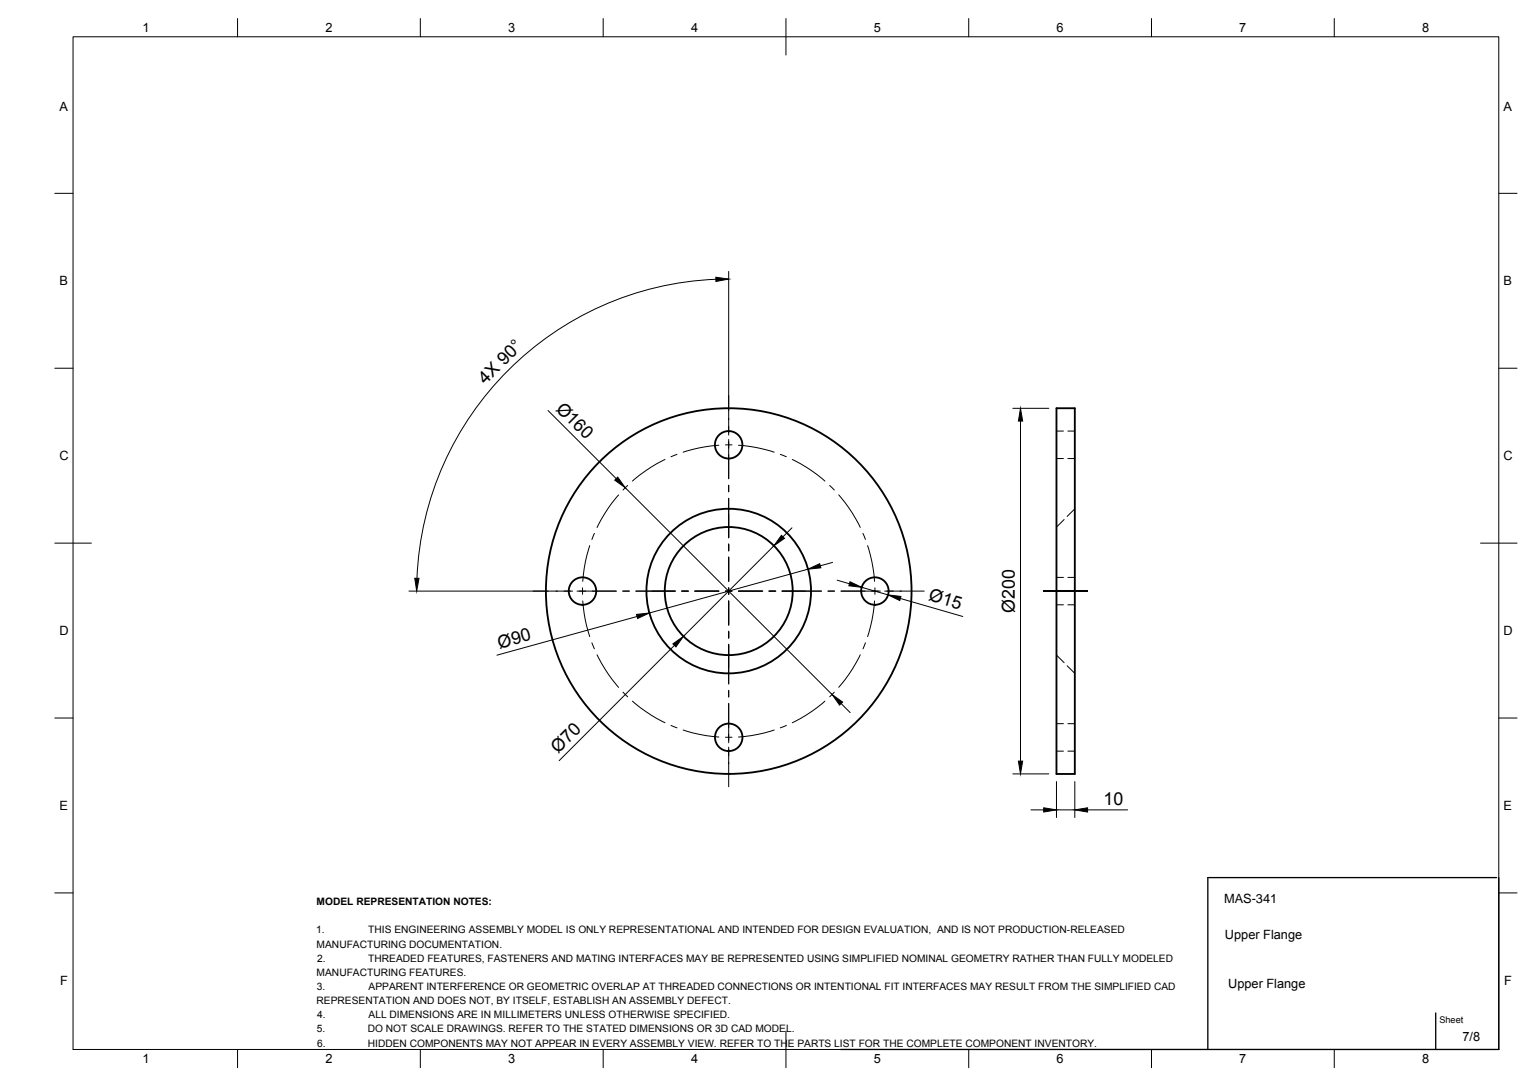
ISO-10303-21;
HEADER;
FILE_DESCRIPTION (('STEP AP214'),
    '1' );
FILE_NAME ('Upper Flange.step',
    '2026-10-08T00:39:10',
    ( '' ),
    ( '' ),
    'SwSTEP 2.0',
    'SolidWorks 2025',
    '' );
FILE_SCHEMA (( 'AUTOMOTIVE_DESIGN' ));
ENDSEC;

DATA;
#46=DIRECTION ( 'NONE',  ( 0.000000000000000000, 1.000000000000000000, 0.000000000000000000 ) ) ;
#104=VECTOR ( 'NONE', #2637, 1000.000000000000000 ) ;
#106=FACE_OUTER_BOUND ( 'NONE', #19908, .T. ) ;
#339=FACE_OUTER_BOUND ( 'NONE', #16289, .T. ) ;
#345=VERTEX_POINT ( 'NONE', #11779 ) ;
#367=EDGE_LOOP ( 'NONE', ( #4657, #4676 ) ) ;
#371=VERTEX_POINT ( 'NONE', #9014 ) ;
#373=ADVANCED_FACE ( 'NONE', ( #2893 ), #13929, .F. ) ;
#378=DIRECTION ( 'NONE',  ( -0.000000000000000000, -1.000000000000000000, -0.000000000000000000 ) ) ;
#387=CARTESIAN_POINT ( 'NONE',  ( -109.9999999999983515, 285.0000000000000568, 92.50000000000004263 ) ) ;
#392=ORIENTED_EDGE ( 'NONE', *, *, #15866, .T. ) ;
#411=DIRECTION ( 'NONE',  ( 0.000000000000000000, 0.000000000000000000, -1.000000000000000000 ) ) ;
#419=PLANE ( 'NONE',  #4671 ) ;
#422=CARTESIAN_POINT ( 'NONE',  ( -110.0000000000000142, 285.0000000000000568, -82.50000000000001421 ) ) ;
#511=DIRECTION ( 'NONE',  ( 0.000000000000000000, 1.000000000000000000, 0.000000000000000000 ) ) ;
#541=VERTEX_POINT ( 'NONE', #10137 ) ;
#552=EDGE_LOOP ( 'NONE', ( #7577, #5145, #8695, #8498 ) ) ;
#564=DIRECTION ( 'NONE',  ( -0.000000000000000000, -1.000000000000000000, -0.000000000000000000 ) ) ;
#565=DIRECTION ( 'NONE',  ( -0.000000000000000000, -1.000000000000000000, -0.000000000000000000 ) ) ;
#609=CIRCLE ( 'NONE', #7461, 34.99999999999997868 ) ;
#638=ORIENTED_EDGE ( 'NONE', *, *, #4760, .F. ) ;
#642=CARTESIAN_POINT ( 'NONE',  ( -110.0000000000000142, 275.0000000000000000, 5.000000000000000888 ) ) ;
#648=VERTEX_POINT ( 'NONE', #17925 ) ;
#660=EDGE_CURVE ( 'NONE', #17410, #15549, #8916, .T. ) ;
#668=PRODUCT_DEFINITION_CONTEXT ( 'detailed design', #4634, 'design' ) ;
#671=PRODUCT_DEFINITION_FORMATION_WITH_SPECIFIED_SOURCE ( 'ANY', '', #15700, .NOT_KNOWN. ) ;
#676=ORIENTED_EDGE ( 'NONE', *, *, #9749, .T. ) ;
#775=AXIS2_PLACEMENT_3D ( 'NONE', #10807, #9387, #14194 ) ;
#811=CIRCLE ( 'NONE', #18457, 99.99999999999997158 ) ;
#815=CARTESIAN_POINT ( 'NONE',  ( -29.99999999999887379, 275.0000000000000000, 4.999999999999158007 ) ) ;
#883=ORIENTED_EDGE ( 'NONE', *, *, #14292, .T. ) ;
#1036=AXIS2_PLACEMENT_3D ( 'NONE', #12711, #18869, #17440 ) ;
#1094=EDGE_CURVE ( 'NONE', #541, #1941, #19405, .T. ) ;
#1096=DIRECTION ( 'NONE',  ( -0.000000000000000000, -1.000000000000000000, -0.000000000000000000 ) ) ;
#1099=EDGE_CURVE ( 'NONE', #16204, #18358, #3152, .T. ) ;
#1141=EDGE_LOOP ( 'NONE', ( #1644, #11755 ) ) ;
#1161=ORIENTED_EDGE ( 'NONE', *, *, #1765, .F. ) ;
#1186=MANIFOLD_SOLID_BREP ( 'Chamfer1', #7388 ) ;
#1187=VERTEX_POINT ( 'NONE', #19014 ) ;
#1382=VECTOR ( 'NONE', #13012, 1000.000000000000000 ) ;
#1402=EDGE_LOOP ( 'NONE', ( #11155, #2446, #12157, #14344 ) ) ;
#1517=AXIS2_PLACEMENT_3D ( 'NONE', #15686, #15576, #15255 ) ;
#1539=ORIENTED_EDGE ( 'NONE', *, *, #14292, .F. ) ;
#1564=CARTESIAN_POINT ( 'NONE',  ( -29.99999999999887379, 285.0000000000000568, 4.999999999999158007 ) ) ;
#1644=ORIENTED_EDGE ( 'NONE', *, *, #9146, .T. ) ;
#1750=CARTESIAN_POINT ( 'NONE',  ( -110.0000000000000142, 285.0000000000000568, 5.000000000000000888 ) ) ;
#1765=EDGE_CURVE ( 'NONE', #16453, #5784, #19740, .T. ) ;
#1868=FACE_BOUND ( 'NONE', #4582, .T. ) ;
#1922=FILL_AREA_STYLE ('',( #15934 ) ) ;
#1941=VERTEX_POINT ( 'NONE', #1953 ) ;
#1953=CARTESIAN_POINT ( 'NONE',  ( -110.0000000000000142, 285.0000000000000568, 50.00000000000000000 ) ) ;
#1971=PRODUCT_CONTEXT ( 'NONE', #13758, 'mechanical' ) ;
#1976=FACE_OUTER_BOUND ( 'NONE', #19531, .T. ) ;
#2046=DIRECTION ( 'NONE',  ( 0.000000000000000000, 0.000000000000000000, 1.000000000000000000 ) ) ;
#2093=COLOUR_RGB ( '', 0.40784314, 0.44705882, 0.49803922) ;
#2165=FACE_BOUND ( 'NONE', #2281, .T. ) ;
#2279=FACE_BOUND ( 'NONE', #10646, .T. ) ;
#2281=EDGE_LOOP ( 'NONE', ( #15820, #17001 ) ) ;
#2293=CYLINDRICAL_SURFACE ( 'NONE', #10703, 99.99999999999997158 ) ;
#2388=EDGE_CURVE ( 'NONE', #13281, #345, #2976, .T. ) ;
#2425=LINE ( 'NONE', #2517, #20217 ) ;
#2437=ORIENTED_EDGE ( 'NONE', *, *, #13531, .F. ) ;
#2446=ORIENTED_EDGE ( 'NONE', *, *, #11970, .F. ) ;
#2479=EDGE_LOOP ( 'NONE', ( #13804, #13370 ) ) ;
#2509=CONICAL_SURFACE ( 'NONE', #10337, 34.99999999999997868, 0.7853981633974521648 ) ;
#2517=CARTESIAN_POINT ( 'NONE',  ( -109.9999999999983515, 285.0000000000000568, 92.50000000000004263 ) ) ;
#2529=CARTESIAN_POINT ( 'NONE',  ( -29.99999999999887379, 285.0000000000000568, -2.500000000000847766 ) ) ;
#2548=CARTESIAN_POINT ( 'NONE',  ( -29.99999999999887379, 275.0000000000000000, 12.49999999999916511 ) ) ;
#2559=ORIENTED_EDGE ( 'NONE', *, *, #8365, .F. ) ;
#2600=ORIENTED_EDGE ( 'NONE', *, *, #11970, .T. ) ;
#2618=DIRECTION ( 'NONE',  ( 0.000000000000000000, 1.000000000000000000, 0.000000000000000000 ) ) ;
#2624=CIRCLE ( 'NONE', #17073, 7.500000000000020428 ) ;
#2637=DIRECTION ( 'NONE',  ( 0.000000000000000000, 0.7071067811865447972, 0.7071067811865502373 ) ) ;
#2651=CARTESIAN_POINT ( 'NONE',  ( -109.9999999999983515, 285.0000000000000568, 85.00000000000001421 ) ) ;
#2681=LINE ( 'NONE', #13204, #19215 ) ;
#2712=ORIENTED_EDGE ( 'NONE', *, *, #660, .F. ) ;
#2730=DIRECTION ( 'NONE',  ( 0.000000000000000000, 1.000000000000000000, 0.000000000000000000 ) ) ;
#2793=VERTEX_POINT ( 'NONE', #13529 ) ;
#2814=ORIENTED_EDGE ( 'NONE', *, *, #15802, .T. ) ;
#2893=FACE_OUTER_BOUND ( 'NONE', #3242, .T. ) ;
#2937=AXIS2_PLACEMENT_3D ( 'NONE', #11804, #7124, #5792 ) ;
#2976=CIRCLE ( 'NONE', #4279, 7.500000000000020428 ) ;
#2996=EDGE_LOOP ( 'NONE', ( #14290, #392, #6277, #2437 ) ) ;
#3007=DIRECTION ( 'NONE',  ( -0.000000000000000000, -1.000000000000000000, -0.000000000000000000 ) ) ;
#3152=LINE ( 'NONE', #17171, #15816 ) ;
#3169=CARTESIAN_POINT ( 'NONE',  ( -189.9999999999988916, 285.0000000000000568, 5.000000000000268230 ) ) ;
#3228=VECTOR ( 'NONE', #565, 1000.000000000000000 ) ;
#3242=EDGE_LOOP ( 'NONE', ( #10222, #5250, #13945, #15544 ) ) ;
#3422=( GEOMETRIC_REPRESENTATION_CONTEXT ( 3 ) GLOBAL_UNCERTAINTY_ASSIGNED_CONTEXT ( ( #12118 ) ) GLOBAL_UNIT_ASSIGNED_CONTEXT ( ( #18810, #17376, #7944 ) ) REPRESENTATION_CONTEXT ( 'NONE', 'WORKASPACE' ) );
#3444=VERTEX_POINT ( 'NONE', #4937 ) ;
#3478=CARTESIAN_POINT ( 'NONE',  ( -110.0000000000000142, 285.0000000000000568, 5.000000000000000888 ) ) ;
#3524=PRODUCT_DEFINITION ( 'UNKNOWN', '', #671, #668 ) ;
#3532=CARTESIAN_POINT ( 'NONE',  ( -110.0000000000000142, 285.0000000000000568, -67.49999999999997158 ) ) ;
#3541=VECTOR ( 'NONE', #5142, 1000.000000000000000 ) ;
#3710=CIRCLE ( 'NONE', #16124, 7.500000000000007105 ) ;
#3768=CARTESIAN_POINT ( 'NONE',  ( -110.0000000000000142, 275.0000000000000568, 5.000000000000000888 ) ) ;
#3770=LINE ( 'NONE', #5415, #5109 ) ;
#3771=FACE_OUTER_BOUND ( 'NONE', #14291, .T. ) ;
#3784=FACE_BOUND ( 'NONE', #10674, .T. ) ;
#3787=DIRECTION ( 'NONE',  ( 0.000000000000000000, 1.000000000000000000, 0.000000000000000000 ) ) ;
#3799=DIRECTION ( 'NONE',  ( 0.000000000000000000, 1.000000000000000000, 0.000000000000000000 ) ) ;
#3801=EDGE_LOOP ( 'NONE', ( #2712, #9678, #676, #12389 ) ) ;
#3870=EDGE_CURVE ( 'NONE', #7406, #3444, #2624, .T. ) ;
#3909=DIRECTION ( 'NONE',  ( 0.000000000000000000, 0.000000000000000000, 1.000000000000000000 ) ) ;
#4075=CARTESIAN_POINT ( 'NONE',  ( -110.0000000000000142, 275.0000000000000568, 5.000000000000000888 ) ) ;
#4084=AXIS2_PLACEMENT_3D ( 'NONE', #19276, #11584, #14458 ) ;
#4118=EDGE_CURVE ( 'NONE', #16923, #16598, #15430, .T. ) ;
#4156=DIRECTION ( 'NONE',  ( 0.000000000000000000, 0.000000000000000000, 1.000000000000000000 ) ) ;
#4173=ORIENTED_EDGE ( 'NONE', *, *, #4760, .T. ) ;
#4279=AXIS2_PLACEMENT_3D ( 'NONE', #10191, #13349, #11809 ) ;
#4294=CARTESIAN_POINT ( 'NONE',  ( -110.0000000000000142, 285.0000000000000568, 5.000000000000000888 ) ) ;
#4344=CIRCLE ( 'NONE', #13475, 45.00000000000001421 ) ;
#4536=CARTESIAN_POINT ( 'NONE',  ( -109.9999999999983515, 285.0000000000000568, 85.00000000000001421 ) ) ;
#4582=EDGE_LOOP ( 'NONE', ( #7260, #4173 ) ) ;
#4624=ORIENTED_EDGE ( 'NONE', *, *, #12645, .F. ) ;
#4634=APPLICATION_CONTEXT ( 'automotive_design' ) ;
#4649=CARTESIAN_POINT ( 'NONE',  ( -189.9999999999988916, 285.0000000000000568, 5.000000000000268230 ) ) ;
#4657=ORIENTED_EDGE ( 'NONE', *, *, #12645, .T. ) ;
#4671=AXIS2_PLACEMENT_3D ( 'NONE', #1750, #7984, #18010 ) ;
#4676=ORIENTED_EDGE ( 'NONE', *, *, #16658, .T. ) ;
#4760=EDGE_CURVE ( 'NONE', #19487, #18358, #3710, .T. ) ;
#4937=CARTESIAN_POINT ( 'NONE',  ( -110.0000000000000142, 275.0000000000000000, -82.50000000000001421 ) ) ;
#4981=ADVANCED_FACE ( 'NONE', ( #17188 ), #5113, .F. ) ;
#4983=CARTESIAN_POINT ( 'NONE',  ( -110.0000000000000142, 275.0000000000000000, -94.99999999999997158 ) ) ;
#5040=LINE ( 'NONE', #422, #3541 ) ;
#5097=SURFACE_STYLE_USAGE ( .BOTH. , #11114 ) ;
#5109=VECTOR ( 'NONE', #20024, 1000.000000000000000 ) ;
#5113=CYLINDRICAL_SURFACE ( 'NONE', #14164, 7.500000000000003553 ) ;
#5142=DIRECTION ( 'NONE',  ( -0.000000000000000000, -1.000000000000000000, -0.000000000000000000 ) ) ;
#5145=ORIENTED_EDGE ( 'NONE', *, *, #4118, .T. ) ;
#5160=CIRCLE ( 'NONE', #19199, 7.500000000000020428 ) ;
#5190=ORIENTED_EDGE ( 'NONE', *, *, #9146, .F. ) ;
#5191=ORIENTED_EDGE ( 'NONE', *, *, #3870, .F. ) ;
#5248=PLANE ( 'NONE',  #16148 ) ;
#5250=ORIENTED_EDGE ( 'NONE', *, *, #7228, .T. ) ;
#5305=DIRECTION ( 'NONE',  ( 0.000000000000000000, 0.000000000000000000, -1.000000000000000000 ) ) ;
#5308=CIRCLE ( 'NONE', #16727, 34.99999999999997868 ) ;
#5326=FACE_OUTER_BOUND ( 'NONE', #1402, .T. ) ;
#5415=CARTESIAN_POINT ( 'NONE',  ( -110.0000000000000000, 285.0000000000000568, 104.9999999999999858 ) ) ;
#5449=DIRECTION ( 'NONE',  ( 0.000000000000000000, 1.000000000000000000, 0.000000000000000000 ) ) ;
#5496=CARTESIAN_POINT ( 'NONE',  ( -110.0000000000000000, 285.0000000000000568, 104.9999999999999858 ) ) ;
#5523=DIRECTION ( 'NONE',  ( 0.000000000000000000, 1.000000000000000000, 0.000000000000000000 ) ) ;
#5549=CIRCLE ( 'NONE', #2937, 99.99999999999997158 ) ;
#5562=DIRECTION ( 'NONE',  ( 0.000000000000000000, 0.000000000000000000, 1.000000000000000000 ) ) ;
#5573=AXIS2_PLACEMENT_3D ( 'NONE', #19141, #7774, #411 ) ;
#5721=DIRECTION ( 'NONE',  ( 0.000000000000000000, 0.000000000000000000, 1.000000000000000000 ) ) ;
#5784=VERTEX_POINT ( 'NONE', #12929 ) ;
#5792=DIRECTION ( 'NONE',  ( 0.000000000000000000, 0.000000000000000000, 1.000000000000000000 ) ) ;
#6058=CARTESIAN_POINT ( 'NONE',  ( -109.9999999999983515, 275.0000000000000000, 85.00000000000001421 ) ) ;
#6078=FACE_OUTER_BOUND ( 'NONE', #14539, .T. ) ;
#6091=ORIENTED_EDGE ( 'NONE', *, *, #11766, .T. ) ;
#6231=AXIS2_PLACEMENT_3D ( 'NONE', #4536, #3007, #7696 ) ;
#6277=ORIENTED_EDGE ( 'NONE', *, *, #13465, .F. ) ;
#6401=ORIENTED_EDGE ( 'NONE', *, *, #12375, .T. ) ;
#6416=CARTESIAN_POINT ( 'NONE',  ( -110.0000000000000142, 275.0000000000000000, -29.99999999999998224 ) ) ;
#6474=ORIENTED_EDGE ( 'NONE', *, *, #11766, .F. ) ;
#6485=VECTOR ( 'NONE', #18378, 1000.000000000000000 ) ;
#6580=ORIENTED_EDGE ( 'NONE', *, *, #4118, .F. ) ;
#6660=CYLINDRICAL_SURFACE ( 'NONE', #17825, 7.500000000000020428 ) ;
#6747=DIRECTION ( 'NONE',  ( -0.000000000000000000, -1.000000000000000000, -0.000000000000000000 ) ) ;
#6754=DIRECTION ( 'NONE',  ( 0.000000000000000000, 0.000000000000000000, 1.000000000000000000 ) ) ;
#6903=CARTESIAN_POINT ( 'NONE',  ( -189.9999999999988916, 275.0000000000000000, 5.000000000000268230 ) ) ;
#7007=EDGE_CURVE ( 'NONE', #16598, #16923, #19661, .T. ) ;
#7072=AXIS2_PLACEMENT_3D ( 'NONE', #7625, #20211, #12433 ) ;
#7093=EDGE_CURVE ( 'NONE', #16460, #371, #5308, .T. ) ;
#7124=DIRECTION ( 'NONE',  ( 0.000000000000000000, 1.000000000000000000, 0.000000000000000000 ) ) ;
#7142=LINE ( 'NONE', #13361, #104 ) ;
#7221=DIRECTION ( 'NONE',  ( -0.000000000000000000, -1.000000000000000000, -0.000000000000000000 ) ) ;
#7228=EDGE_CURVE ( 'NONE', #11511, #19487, #13104, .T. ) ;
#7231=CYLINDRICAL_SURFACE ( 'NONE', #16232, 7.500000000000003553 ) ;
#7260=ORIENTED_EDGE ( 'NONE', *, *, #17492, .T. ) ;
#7303=DIRECTION ( 'NONE',  ( 0.000000000000000000, 1.000000000000000000, 0.000000000000000000 ) ) ;
#7388=CLOSED_SHELL ( 'NONE', ( #11718, #16256, #18901, #373, #9034, #19166, #15927, #14415, #17648, #15605, #19262, #10516, #4981, #16900 ) ) ;
#7406=VERTEX_POINT ( 'NONE', #11049 ) ;
#7461=AXIS2_PLACEMENT_3D ( 'NONE', #15313, #9283, #14193 ) ;
#7525=CARTESIAN_POINT ( 'NONE',  ( -189.9999999999988916, 285.0000000000000568, -2.499999999999734879 ) ) ;
#7577=ORIENTED_EDGE ( 'NONE', *, *, #9978, .F. ) ;
#7617=ORIENTED_EDGE ( 'NONE', *, *, #18627, .T. ) ;
#7625=CARTESIAN_POINT ( 'NONE',  ( -29.99999999999887379, 285.0000000000000568, 4.999999999999158007 ) ) ;
#7672=CYLINDRICAL_SURFACE ( 'NONE', #11118, 99.99999999999997158 ) ;
#7696=DIRECTION ( 'NONE',  ( 0.000000000000000000, 0.000000000000000000, -1.000000000000000000 ) ) ;
#7711=CIRCLE ( 'NONE', #7072, 7.500000000000007105 ) ;
#7774=DIRECTION ( 'NONE',  ( -0.000000000000000000, -1.000000000000000000, -0.000000000000000000 ) ) ;
#7779=DIRECTION ( 'NONE',  ( 0.000000000000000000, 1.000000000000000000, 0.000000000000000000 ) ) ;
#7812=CIRCLE ( 'NONE', #9765, 7.500000000000020428 ) ;
#7823=ORIENTED_EDGE ( 'NONE', *, *, #9670, .T. ) ;
#7851=UNCERTAINTY_MEASURE_WITH_UNIT (LENGTH_MEASURE( 1.000000000000000082E-05 ), #10342, 'distance_accuracy_value', 'NONE');
#7862=ORIENTED_EDGE ( 'NONE', *, *, #18627, .F. ) ;
#7910=DIRECTION ( 'NONE',  ( 0.000000000000000000, 0.000000000000000000, 1.000000000000000000 ) ) ;
#7921=EDGE_LOOP ( 'NONE', ( #16328, #14035, #14267, #13897 ) ) ;
#7944=( NAMED_UNIT ( * ) SI_UNIT ( $, .STERADIAN. ) SOLID_ANGLE_UNIT ( ) );
#7972=CIRCLE ( 'NONE', #17471, 7.500000000000007105 ) ;
#7984=DIRECTION ( 'NONE',  ( 0.000000000000000000, 1.000000000000000000, 0.000000000000000000 ) ) ;
#8020=ORIENTED_EDGE ( 'NONE', *, *, #7228, .F. ) ;
#8026=LINE ( 'NONE', #11403, #17967 ) ;
#8069=AXIS2_PLACEMENT_3D ( 'NONE', #6058, #7779, #16891 ) ;
#8098=FACE_BOUND ( 'NONE', #367, .T. ) ;
#8114=CONICAL_SURFACE ( 'NONE', #13019, 34.99999999999997868, 0.7853981633974521648 ) ;
#8170=DIRECTION ( 'NONE',  ( -0.000000000000000000, -1.000000000000000000, -0.000000000000000000 ) ) ;
#8198=ORIENTED_EDGE ( 'NONE', *, *, #16363, .F. ) ;
#8326=DIRECTION ( 'NONE',  ( 0.000000000000000000, 1.000000000000000000, 0.000000000000000000 ) ) ;
#8365=EDGE_CURVE ( 'NONE', #17410, #5784, #3770, .T. ) ;
#8374=DIRECTION ( 'NONE',  ( 0.000000000000000000, 0.000000000000000000, 1.000000000000000000 ) ) ;
#8389=FACE_BOUND ( 'NONE', #2479, .T. ) ;
#8416=CARTESIAN_POINT ( 'NONE',  ( 0.000000000000000000, 0.000000000000000000, 0.000000000000000000 ) ) ;
#8439=CIRCLE ( 'NONE', #20192, 7.500000000000020428 ) ;
#8498=ORIENTED_EDGE ( 'NONE', *, *, #15802, .F. ) ;
#8507=CARTESIAN_POINT ( 'NONE',  ( -110.0000000000000142, 275.0000000000000000, 5.000000000000000888 ) ) ;
#8518=CARTESIAN_POINT ( 'NONE',  ( -110.0000000000000142, 285.0000000000000568, -94.99999999999997158 ) ) ;
#8669=CARTESIAN_POINT ( 'NONE',  ( -110.0000000000000142, 285.0000000000000568, 5.000000000000000888 ) ) ;
#8694=ADVANCED_BREP_SHAPE_REPRESENTATION ( '', ( #1186, #18639 ), #14384 ) ;
#8695=ORIENTED_EDGE ( 'NONE', *, *, #17533, .T. ) ;
#8720=DIRECTION ( 'NONE',  ( 0.000000000000000000, 0.000000000000000000, 1.000000000000000000 ) ) ;
#8736=CIRCLE ( 'NONE', #12673, 7.500000000000007105 ) ;
#8757=ORIENTED_EDGE ( 'NONE', *, *, #18025, .T. ) ;
#8786=CARTESIAN_POINT ( 'NONE',  ( -109.9999999999983515, 285.0000000000000568, 85.00000000000001421 ) ) ;
#8905=DIRECTION ( 'NONE',  ( -0.000000000000000000, -1.000000000000000000, -0.000000000000000000 ) ) ;
#8916=CIRCLE ( 'NONE', #19081, 99.99999999999997158 ) ;
#8951=LINE ( 'NONE', #7525, #6485 ) ;
#8961=ORIENTED_EDGE ( 'NONE', *, *, #17533, .F. ) ;
#8992=DIRECTION ( 'NONE',  ( 0.000000000000000000, 0.000000000000000000, 1.000000000000000000 ) ) ;
#9014=CARTESIAN_POINT ( 'NONE',  ( -110.0000000000000142, 275.0000000000000000, 39.99999999999997868 ) ) ;
#9034=ADVANCED_FACE ( 'NONE', ( #3771 ), #6660, .F. ) ;
#9044=DIRECTION ( 'NONE',  ( 0.000000000000000000, 0.000000000000000000, 1.000000000000000000 ) ) ;
#9091=VERTEX_POINT ( 'NONE', #16168 ) ;
#9146=EDGE_CURVE ( 'NONE', #15549, #17410, #811, .T. ) ;
#9179=ORIENTED_EDGE ( 'NONE', *, *, #7007, .F. ) ;
#9283=DIRECTION ( 'NONE',  ( 0.000000000000000000, 1.000000000000000000, 0.000000000000000000 ) ) ;
#9387=DIRECTION ( 'NONE',  ( -0.000000000000000000, -1.000000000000000000, -0.000000000000000000 ) ) ;
#9625=CARTESIAN_POINT ( 'NONE',  ( -110.0000000000000142, 275.0000000000000568, -29.99999999999998224 ) ) ;
#9634=SHAPE_DEFINITION_REPRESENTATION ( #10940, #16185 ) ;
#9660=EDGE_CURVE ( 'NONE', #1187, #15465, #7812, .T. ) ;
#9670=EDGE_CURVE ( 'NONE', #15465, #9091, #2425, .T. ) ;
#9678=ORIENTED_EDGE ( 'NONE', *, *, #8365, .T. ) ;
#9749=EDGE_CURVE ( 'NONE', #5784, #16453, #5549, .T. ) ;
#9765=AXIS2_PLACEMENT_3D ( 'NONE', #15085, #14887, #13343 ) ;
#9787=CARTESIAN_POINT ( 'NONE',  ( -110.0000000000000142, 285.0000000000000568, -94.99999999999997158 ) ) ;
#9950=CARTESIAN_POINT ( 'NONE',  ( -29.99999999999887379, 285.0000000000000568, 12.49999999999916511 ) ) ;
#9978=EDGE_CURVE ( 'NONE', #16923, #2793, #8026, .T. ) ;
#10033=DIRECTION ( 'NONE',  ( 0.000000000000000000, 0.000000000000000000, 1.000000000000000000 ) ) ;
#10053=DIRECTION ( 'NONE',  ( 0.000000000000000000, 1.000000000000000000, 0.000000000000000000 ) ) ;
#10137=CARTESIAN_POINT ( 'NONE',  ( -110.0000000000000142, 285.0000000000000568, -40.00000000000000711 ) ) ;
#10191=CARTESIAN_POINT ( 'NONE',  ( -110.0000000000000142, 285.0000000000000568, -75.00000000000000000 ) ) ;
#10222=ORIENTED_EDGE ( 'NONE', *, *, #16363, .T. ) ;
#10337=AXIS2_PLACEMENT_3D ( 'NONE', #4075, #5523, #16175 ) ;
#10342=( LENGTH_UNIT ( ) NAMED_UNIT ( * ) SI_UNIT ( .MILLI., .METRE. ) );
#10365=ORIENTED_EDGE ( 'NONE', *, *, #1765, .T. ) ;
#10516=ADVANCED_FACE ( 'NONE', ( #16757 ), #16664, .F. ) ;
#10542=( NAMED_UNIT ( * ) PLANE_ANGLE_UNIT ( ) SI_UNIT ( $, .RADIAN. ) );
#10617=EDGE_LOOP ( 'NONE', ( #19575, #18268, #11605, #8961 ) ) ;
#10646=EDGE_LOOP ( 'NONE', ( #12756, #2814 ) ) ;
#10672=CIRCLE ( 'NONE', #8069, 7.500000000000020428 ) ;
#10674=EDGE_LOOP ( 'NONE', ( #8198, #1539 ) ) ;
#10703=AXIS2_PLACEMENT_3D ( 'NONE', #16402, #19469, #11680 ) ;
#10706=DIRECTION ( 'NONE',  ( 0.000000000000000000, 1.000000000000000000, 0.000000000000000000 ) ) ;
#10738=FACE_OUTER_BOUND ( 'NONE', #3801, .T. ) ;
#10807=CARTESIAN_POINT ( 'NONE',  ( -110.0000000000000142, 285.0000000000000568, 5.000000000000000888 ) ) ;
#10857=ORIENTED_EDGE ( 'NONE', *, *, #1094, .T. ) ;
#10940=PRODUCT_DEFINITION_SHAPE ( 'NONE', 'NONE',  #3524 ) ;
#11011=SURFACE_STYLE_FILL_AREA ( #1922 ) ;
#11049=CARTESIAN_POINT ( 'NONE',  ( -110.0000000000000142, 275.0000000000000000, -67.49999999999997158 ) ) ;
#11114=SURFACE_SIDE_STYLE ('',( #11011 ) ) ;
#11118=AXIS2_PLACEMENT_3D ( 'NONE', #13911, #20156, #19747 ) ;
#11155=ORIENTED_EDGE ( 'NONE', *, *, #15866, .F. ) ;
#11161=ORIENTED_EDGE ( 'NONE', *, *, #1099, .T. ) ;
#11195=LINE ( 'NONE', #3532, #3228 ) ;
#11403=CARTESIAN_POINT ( 'NONE',  ( -189.9999999999988916, 285.0000000000000568, 12.50000000000027178 ) ) ;
#11474=DIRECTION ( 'NONE',  ( 0.000000000000000000, -0.000000000000000000, 1.000000000000000000 ) ) ;
#11511=VERTEX_POINT ( 'NONE', #16485 ) ;
#11584=DIRECTION ( 'NONE',  ( -0.000000000000000000, -1.000000000000000000, -0.000000000000000000 ) ) ;
#11605=ORIENTED_EDGE ( 'NONE', *, *, #12964, .F. ) ;
#11678=CARTESIAN_POINT ( 'NONE',  ( -189.9999999999988916, 275.0000000000000000, 5.000000000000268230 ) ) ;
#11680=DIRECTION ( 'NONE',  ( 0.000000000000000000, 0.000000000000000000, -1.000000000000000000 ) ) ;
#11718=ADVANCED_FACE ( 'NONE', ( #17600 ), #8114, .F. ) ;
#11743=ORIENTED_EDGE ( 'NONE', *, *, #18025, .F. ) ;
#11755=ORIENTED_EDGE ( 'NONE', *, *, #660, .T. ) ;
#11765=DIRECTION ( 'NONE',  ( 0.000000000000000000, 0.000000000000000000, 1.000000000000000000 ) ) ;
#11766=EDGE_CURVE ( 'NONE', #3444, #7406, #17966, .T. ) ;
#11776=( NAMED_UNIT ( * ) SI_UNIT ( $, .STERADIAN. ) SOLID_ANGLE_UNIT ( ) );
#11779=CARTESIAN_POINT ( 'NONE',  ( -110.0000000000000142, 285.0000000000000568, -67.49999999999997158 ) ) ;
#11804=CARTESIAN_POINT ( 'NONE',  ( -110.0000000000000142, 275.0000000000000000, 5.000000000000000888 ) ) ;
#11809=DIRECTION ( 'NONE',  ( 0.000000000000000000, 0.000000000000000000, 1.000000000000000000 ) ) ;
#11970=EDGE_CURVE ( 'NONE', #371, #16460, #609, .T. ) ;
#12024=CIRCLE ( 'NONE', #14329, 7.500000000000003553 ) ;
#12118=UNCERTAINTY_MEASURE_WITH_UNIT (LENGTH_MEASURE( 1.000000000000000082E-05 ), #18810, 'distance_accuracy_value', 'NONE');
#12157=ORIENTED_EDGE ( 'NONE', *, *, #13531, .T. ) ;
#12205=EDGE_CURVE ( 'NONE', #345, #13281, #15261, .T. ) ;
#12375=EDGE_CURVE ( 'NONE', #15549, #16453, #17377, .T. ) ;
#12389=ORIENTED_EDGE ( 'NONE', *, *, #12375, .F. ) ;
#12433=DIRECTION ( 'NONE',  ( 0.000000000000000000, 0.000000000000000000, 1.000000000000000000 ) ) ;
#12437=ORIENTED_EDGE ( 'NONE', *, *, #13465, .T. ) ;
#12496=DIRECTION ( 'NONE',  ( 0.000000000000000000, 1.000000000000000000, 0.000000000000000000 ) ) ;
#12645=EDGE_CURVE ( 'NONE', #648, #9091, #8439, .T. ) ;
#12650=PRESENTATION_STYLE_ASSIGNMENT (( #5097 ) ) ;
#12673=AXIS2_PLACEMENT_3D ( 'NONE', #20004, #2730, #4156 ) ;
#12689=LINE ( 'NONE', #9625, #19051 ) ;
#12711=CARTESIAN_POINT ( 'NONE',  ( -189.9999999999988916, 285.0000000000000568, 5.000000000000268230 ) ) ;
#12756=ORIENTED_EDGE ( 'NONE', *, *, #12964, .T. ) ;
#12808=FACE_BOUND ( 'NONE', #14165, .T. ) ;
#12877=DIRECTION ( 'NONE',  ( 0.000000000000000000, 1.000000000000000000, 0.000000000000000000 ) ) ;
#12901=VERTEX_POINT ( 'NONE', #17246 ) ;
#12929=CARTESIAN_POINT ( 'NONE',  ( -110.0000000000000000, 275.0000000000000000, 104.9999999999999858 ) ) ;
#12964=EDGE_CURVE ( 'NONE', #12901, #2793, #12024, .T. ) ;
#13012=DIRECTION ( 'NONE',  ( -0.000000000000000000, -1.000000000000000000, -0.000000000000000000 ) ) ;
#13019=AXIS2_PLACEMENT_3D ( 'NONE', #3768, #16064, #2046 ) ;
#13073=DIRECTION ( 'NONE',  ( 0.000000000000000000, 0.000000000000000000, -1.000000000000000000 ) ) ;
#13104=LINE ( 'NONE', #9950, #1382 ) ;
#13162=DIRECTION ( 'NONE',  ( 0.000000000000000000, 0.000000000000000000, 1.000000000000000000 ) ) ;
#13204=CARTESIAN_POINT ( 'NONE',  ( -109.9999999999983515, 285.0000000000000568, 77.50000000000000000 ) ) ;
#13281=VERTEX_POINT ( 'NONE', #15750 ) ;
#13343=DIRECTION ( 'NONE',  ( 0.000000000000000000, 0.000000000000000000, 1.000000000000000000 ) ) ;
#13349=DIRECTION ( 'NONE',  ( 0.000000000000000000, 1.000000000000000000, 0.000000000000000000 ) ) ;
#13352=CARTESIAN_POINT ( 'NONE',  ( -189.9999999999988916, 285.0000000000000568, 5.000000000000268230 ) ) ;
#13361=CARTESIAN_POINT ( 'NONE',  ( -110.0000000000000142, 275.0000000000000568, 39.99999999999997868 ) ) ;
#13370=ORIENTED_EDGE ( 'NONE', *, *, #12205, .F. ) ;
#13465=EDGE_CURVE ( 'NONE', #1941, #541, #4344, .T. ) ;
#13475=AXIS2_PLACEMENT_3D ( 'NONE', #8669, #6747, #13162 ) ;
#13493=STYLED_ITEM ( 'NONE', ( #12650 ), #1186 ) ;
#13500=DIRECTION ( 'NONE',  ( 1.000000000000000000, 0.000000000000000000, 0.000000000000000000 ) ) ;
#13527=AXIS2_PLACEMENT_3D ( 'NONE', #19478, #19968, #8720 ) ;
#13529=CARTESIAN_POINT ( 'NONE',  ( -189.9999999999988916, 275.0000000000000000, 12.50000000000027178 ) ) ;
#13531=EDGE_CURVE ( 'NONE', #371, #1941, #7142, .T. ) ;
#13758=APPLICATION_CONTEXT ( 'automotive_design' ) ;
#13797=AXIS2_PLACEMENT_3D ( 'NONE', #11678, #5449, #3909 ) ;
#13804=ORIENTED_EDGE ( 'NONE', *, *, #2388, .F. ) ;
#13897=ORIENTED_EDGE ( 'NONE', *, *, #16658, .F. ) ;
#13911=CARTESIAN_POINT ( 'NONE',  ( -110.0000000000000142, 285.0000000000000568, 5.000000000000000888 ) ) ;
#13915=CARTESIAN_POINT ( 'NONE',  ( -189.9999999999988916, 285.0000000000000568, -2.499999999999734879 ) ) ;
#13929=CYLINDRICAL_SURFACE ( 'NONE', #1517, 7.500000000000006217 ) ;
#13945=ORIENTED_EDGE ( 'NONE', *, *, #17492, .F. ) ;
#13992=AXIS2_PLACEMENT_3D ( 'NONE', #14714, #12877, #8374 ) ;
#14016=CYLINDRICAL_SURFACE ( 'NONE', #5573, 7.500000000000006217 ) ;
#14035=ORIENTED_EDGE ( 'NONE', *, *, #17056, .T. ) ;
#14164=AXIS2_PLACEMENT_3D ( 'NONE', #3169, #8170, #15650 ) ;
#14165=EDGE_LOOP ( 'NONE', ( #2600, #16528 ) ) ;
#14193=DIRECTION ( 'NONE',  ( 0.000000000000000000, 0.000000000000000000, 1.000000000000000000 ) ) ;
#14194=DIRECTION ( 'NONE',  ( 0.000000000000000000, 0.000000000000000000, 1.000000000000000000 ) ) ;
#14267=ORIENTED_EDGE ( 'NONE', *, *, #17699, .T. ) ;
#14290=ORIENTED_EDGE ( 'NONE', *, *, #7093, .F. ) ;
#14291=EDGE_LOOP ( 'NONE', ( #19424, #7617, #6474, #11743 ) ) ;
#14292=EDGE_CURVE ( 'NONE', #11511, #16204, #7972, .T. ) ;
#14329=AXIS2_PLACEMENT_3D ( 'NONE', #6903, #8326, #5562 ) ;
#14344=ORIENTED_EDGE ( 'NONE', *, *, #1094, .F. ) ;
#14384=( GEOMETRIC_REPRESENTATION_CONTEXT ( 3 ) GLOBAL_UNCERTAINTY_ASSIGNED_CONTEXT ( ( #7851 ) ) GLOBAL_UNIT_ASSIGNED_CONTEXT ( ( #10342, #10542, #11776 ) ) REPRESENTATION_CONTEXT ( 'NONE', 'WORKASPACE' ) );
#14415=ADVANCED_FACE ( 'NONE', ( #1976, #12808, #14747, #1868, #8098, #2279 ), #5248, .F. ) ;
#14458=DIRECTION ( 'NONE',  ( 0.000000000000000000, 0.000000000000000000, -1.000000000000000000 ) ) ;
#14539=EDGE_LOOP ( 'NONE', ( #16719, #7823, #4624, #14649 ) ) ;
#14621=CARTESIAN_POINT ( 'NONE',  ( -110.0000000000000142, 285.0000000000000568, -75.00000000000000000 ) ) ;
#14649=ORIENTED_EDGE ( 'NONE', *, *, #17699, .F. ) ;
#14664=AXIS2_PLACEMENT_3D ( 'NONE', #2651, #1096, #15114 ) ;
#14704=FACE_OUTER_BOUND ( 'NONE', #10617, .T. ) ;
#14714=CARTESIAN_POINT ( 'NONE',  ( -110.0000000000000142, 275.0000000000000000, -75.00000000000000000 ) ) ;
#14747=FACE_BOUND ( 'NONE', #15571, .T. ) ;
#14776=CIRCLE ( 'NONE', #13797, 7.500000000000003553 ) ;
#14838=EDGE_LOOP ( 'NONE', ( #9179, #6580 ) ) ;
#14887=DIRECTION ( 'NONE',  ( 0.000000000000000000, 1.000000000000000000, 0.000000000000000000 ) ) ;
#15085=CARTESIAN_POINT ( 'NONE',  ( -109.9999999999983515, 285.0000000000000568, 85.00000000000001421 ) ) ;
#15098=AXIS2_PLACEMENT_3D ( 'NONE', #4649, #46, #7910 ) ;
#15114=DIRECTION ( 'NONE',  ( 0.000000000000000000, 0.000000000000000000, -1.000000000000000000 ) ) ;
#15235=DIRECTION ( 'NONE',  ( 0.000000000000000000, 1.000000000000000000, 0.000000000000000000 ) ) ;
#15255=DIRECTION ( 'NONE',  ( 0.000000000000000000, 0.000000000000000000, -1.000000000000000000 ) ) ;
#15261=CIRCLE ( 'NONE', #15612, 7.500000000000020428 ) ;
#15313=CARTESIAN_POINT ( 'NONE',  ( -110.0000000000000142, 275.0000000000000000, 5.000000000000000888 ) ) ;
#15315=ORIENTED_EDGE ( 'NONE', *, *, #3870, .T. ) ;
#15367=DIRECTION ( 'NONE',  ( 0.000000000000000000, 0.000000000000000000, 1.000000000000000000 ) ) ;
#15430=CIRCLE ( 'NONE', #15098, 7.500000000000003553 ) ;
#15465=VERTEX_POINT ( 'NONE', #387 ) ;
#15544=ORIENTED_EDGE ( 'NONE', *, *, #1099, .F. ) ;
#15549=VERTEX_POINT ( 'NONE', #8518 ) ;
#15571=EDGE_LOOP ( 'NONE', ( #6091, #15315 ) ) ;
#15576=DIRECTION ( 'NONE',  ( -0.000000000000000000, -1.000000000000000000, -0.000000000000000000 ) ) ;
#15605=ADVANCED_FACE ( 'NONE', ( #339 ), #19367, .F. ) ;
#15612=AXIS2_PLACEMENT_3D ( 'NONE', #16960, #10706, #20121 ) ;
#15650=DIRECTION ( 'NONE',  ( 0.000000000000000000, 0.000000000000000000, -1.000000000000000000 ) ) ;
#15686=CARTESIAN_POINT ( 'NONE',  ( -29.99999999999887379, 285.0000000000000568, 4.999999999999158007 ) ) ;
#15700=PRODUCT ( 'Upper Flange', 'Upper Flange', '', ( #1971 ) ) ;
#15750=CARTESIAN_POINT ( 'NONE',  ( -110.0000000000000142, 285.0000000000000568, -82.50000000000001421 ) ) ;
#15768=FACE_BOUND ( 'NONE', #14838, .T. ) ;
#15802=EDGE_CURVE ( 'NONE', #2793, #12901, #14776, .T. ) ;
#15816=VECTOR ( 'NONE', #378, 1000.000000000000000 ) ;
#15820=ORIENTED_EDGE ( 'NONE', *, *, #9660, .F. ) ;
#15866=EDGE_CURVE ( 'NONE', #16460, #541, #12689, .T. ) ;
#15874=DIRECTION ( 'NONE',  ( 8.659560562354966138E-17, 0.7071067811865447972, -0.7071067811865502373 ) ) ;
#15927=ADVANCED_FACE ( 'NONE', ( #19343, #2165, #8389, #17814, #3784, #15768 ), #419, .T. ) ;
#15928=ORIENTED_EDGE ( 'NONE', *, *, #12205, .T. ) ;
#15934=FILL_AREA_STYLE_COLOUR ( '', #2093 ) ;
#16064=DIRECTION ( 'NONE',  ( 0.000000000000000000, 1.000000000000000000, 0.000000000000000000 ) ) ;
#16124=AXIS2_PLACEMENT_3D ( 'NONE', #815, #3787, #10033 ) ;
#16148=AXIS2_PLACEMENT_3D ( 'NONE', #8507, #3799, #11474 ) ;
#16168=CARTESIAN_POINT ( 'NONE',  ( -109.9999999999983515, 275.0000000000000000, 92.50000000000004263 ) ) ;
#16175=DIRECTION ( 'NONE',  ( 0.000000000000000000, 0.000000000000000000, 1.000000000000000000 ) ) ;
#16185=SHAPE_REPRESENTATION ( 'Upper Flange', ( #18639 ), #14384 ) ;
#16204=VERTEX_POINT ( 'NONE', #2529 ) ;
#16232=AXIS2_PLACEMENT_3D ( 'NONE', #13352, #19321, #5305 ) ;
#16256=ADVANCED_FACE ( 'NONE', ( #14704 ), #7231, .F. ) ;
#16289=EDGE_LOOP ( 'NONE', ( #7862, #15928, #8757, #5191 ) ) ;
#16328=ORIENTED_EDGE ( 'NONE', *, *, #9670, .F. ) ;
#16363=EDGE_CURVE ( 'NONE', #16204, #11511, #7711, .T. ) ;
#16365=DIRECTION ( 'NONE',  ( -0.000000000000000000, -1.000000000000000000, -0.000000000000000000 ) ) ;
#16402=CARTESIAN_POINT ( 'NONE',  ( -110.0000000000000142, 285.0000000000000568, 5.000000000000000888 ) ) ;
#16453=VERTEX_POINT ( 'NONE', #4983 ) ;
#16460=VERTEX_POINT ( 'NONE', #6416 ) ;
#16485=CARTESIAN_POINT ( 'NONE',  ( -29.99999999999887379, 285.0000000000000568, 12.49999999999916511 ) ) ;
#16500=ORIENTED_EDGE ( 'NONE', *, *, #9749, .F. ) ;
#16528=ORIENTED_EDGE ( 'NONE', *, *, #7093, .T. ) ;
#16598=VERTEX_POINT ( 'NONE', #13915 ) ;
#16658=EDGE_CURVE ( 'NONE', #9091, #648, #10672, .T. ) ;
#16664=CYLINDRICAL_SURFACE ( 'NONE', #14664, 7.500000000000020428 ) ;
#16718=DIRECTION ( 'NONE',  ( 0.000000000000000000, 0.000000000000000000, 1.000000000000000000 ) ) ;
#16719=ORIENTED_EDGE ( 'NONE', *, *, #9660, .T. ) ;
#16727=AXIS2_PLACEMENT_3D ( 'NONE', #642, #10053, #11765 ) ;
#16757=FACE_OUTER_BOUND ( 'NONE', #7921, .T. ) ;
#16799=MECHANICAL_DESIGN_GEOMETRIC_PRESENTATION_REPRESENTATION('',(#13493),#3422);
#16891=DIRECTION ( 'NONE',  ( 0.000000000000000000, 0.000000000000000000, 1.000000000000000000 ) ) ;
#16894=EDGE_LOOP ( 'NONE', ( #2559, #5190, #6401, #10365 ) ) ;
#16900=ADVANCED_FACE ( 'NONE', ( #5326 ), #2509, .F. ) ;
#16923=VERTEX_POINT ( 'NONE', #19534 ) ;
#16960=CARTESIAN_POINT ( 'NONE',  ( -110.0000000000000142, 285.0000000000000568, -75.00000000000000000 ) ) ;
#17001=ORIENTED_EDGE ( 'NONE', *, *, #17056, .F. ) ;
#17056=EDGE_CURVE ( 'NONE', #15465, #1187, #5160, .T. ) ;
#17073=AXIS2_PLACEMENT_3D ( 'NONE', #17884, #7303, #16718 ) ;
#17171=CARTESIAN_POINT ( 'NONE',  ( -29.99999999999887379, 285.0000000000000568, -2.500000000000847766 ) ) ;
#17188=FACE_OUTER_BOUND ( 'NONE', #552, .T. ) ;
#17246=CARTESIAN_POINT ( 'NONE',  ( -189.9999999999988916, 275.0000000000000000, -2.499999999999734879 ) ) ;
#17376=( NAMED_UNIT ( * ) PLANE_ANGLE_UNIT ( ) SI_UNIT ( $, .RADIAN. ) );
#17377=LINE ( 'NONE', #9787, #19213 ) ;
#17410=VERTEX_POINT ( 'NONE', #5496 ) ;
#17440=DIRECTION ( 'NONE',  ( 0.000000000000000000, 0.000000000000000000, 1.000000000000000000 ) ) ;
#17471=AXIS2_PLACEMENT_3D ( 'NONE', #1564, #12496, #15367 ) ;
#17492=EDGE_CURVE ( 'NONE', #18358, #19487, #8736, .T. ) ;
#17533=EDGE_CURVE ( 'NONE', #16598, #12901, #8951, .T. ) ;
#17600=FACE_OUTER_BOUND ( 'NONE', #2996, .T. ) ;
#17648=ADVANCED_FACE ( 'NONE', ( #19559 ), #2293, .T. ) ;
#17699=EDGE_CURVE ( 'NONE', #1187, #648, #2681, .T. ) ;
#17814=FACE_OUTER_BOUND ( 'NONE', #1141, .T. ) ;
#17825=AXIS2_PLACEMENT_3D ( 'NONE', #14621, #16365, #13073 ) ;
#17878=CARTESIAN_POINT ( 'NONE',  ( -29.99999999999887379, 275.0000000000000000, -2.500000000000847766 ) ) ;
#17884=CARTESIAN_POINT ( 'NONE',  ( -110.0000000000000142, 275.0000000000000000, -75.00000000000000000 ) ) ;
#17925=CARTESIAN_POINT ( 'NONE',  ( -109.9999999999983515, 275.0000000000000000, 77.50000000000000000 ) ) ;
#17966=CIRCLE ( 'NONE', #13992, 7.500000000000020428 ) ;
#17967=VECTOR ( 'NONE', #564, 1000.000000000000000 ) ;
#18010=DIRECTION ( 'NONE',  ( 0.000000000000000000, -0.000000000000000000, 1.000000000000000000 ) ) ;
#18025=EDGE_CURVE ( 'NONE', #13281, #3444, #5040, .T. ) ;
#18031=DIRECTION ( 'NONE',  ( 0.000000000000000000, 0.000000000000000000, 1.000000000000000000 ) ) ;
#18268=ORIENTED_EDGE ( 'NONE', *, *, #9978, .T. ) ;
#18358=VERTEX_POINT ( 'NONE', #17878 ) ;
#18378=DIRECTION ( 'NONE',  ( -0.000000000000000000, -1.000000000000000000, -0.000000000000000000 ) ) ;
#18457=AXIS2_PLACEMENT_3D ( 'NONE', #3478, #511, #6754 ) ;
#18554=CYLINDRICAL_SURFACE ( 'NONE', #6231, 7.500000000000020428 ) ;
#18571=CARTESIAN_POINT ( 'NONE',  ( -109.9999999999983515, 275.0000000000000000, 85.00000000000001421 ) ) ;
#18627=EDGE_CURVE ( 'NONE', #345, #7406, #11195, .T. ) ;
#18639=AXIS2_PLACEMENT_3D ( 'NONE', #8416, #18031, #13500 ) ;
#18810=( LENGTH_UNIT ( ) NAMED_UNIT ( * ) SI_UNIT ( .MILLI., .METRE. ) );
#18869=DIRECTION ( 'NONE',  ( 0.000000000000000000, 1.000000000000000000, 0.000000000000000000 ) ) ;
#18901=ADVANCED_FACE ( 'NONE', ( #6078 ), #18554, .F. ) ;
#18911=DIRECTION ( 'NONE',  ( -0.000000000000000000, -1.000000000000000000, -0.000000000000000000 ) ) ;
#19014=CARTESIAN_POINT ( 'NONE',  ( -109.9999999999983515, 285.0000000000000568, 77.50000000000000000 ) ) ;
#19051=VECTOR ( 'NONE', #15874, 1000.000000000000000 ) ;
#19081=AXIS2_PLACEMENT_3D ( 'NONE', #4294, #15235, #8992 ) ;
#19141=CARTESIAN_POINT ( 'NONE',  ( -29.99999999999887379, 285.0000000000000568, 4.999999999999158007 ) ) ;
#19166=ADVANCED_FACE ( 'NONE', ( #10738 ), #7672, .T. ) ;
#19199=AXIS2_PLACEMENT_3D ( 'NONE', #8786, #20034, #5721 ) ;
#19213=VECTOR ( 'NONE', #18911, 1000.000000000000000 ) ;
#19215=VECTOR ( 'NONE', #8905, 1000.000000000000000 ) ;
#19262=ADVANCED_FACE ( 'NONE', ( #106 ), #14016, .F. ) ;
#19276=CARTESIAN_POINT ( 'NONE',  ( -110.0000000000000142, 285.0000000000000568, -75.00000000000000000 ) ) ;
#19321=DIRECTION ( 'NONE',  ( -0.000000000000000000, -1.000000000000000000, -0.000000000000000000 ) ) ;
#19343=FACE_BOUND ( 'NONE', #19384, .T. ) ;
#19367=CYLINDRICAL_SURFACE ( 'NONE', #4084, 7.500000000000020428 ) ;
#19384=EDGE_LOOP ( 'NONE', ( #12437, #10857 ) ) ;
#19405=CIRCLE ( 'NONE', #775, 45.00000000000001421 ) ;
#19424=ORIENTED_EDGE ( 'NONE', *, *, #2388, .T. ) ;
#19469=DIRECTION ( 'NONE',  ( -0.000000000000000000, -1.000000000000000000, -0.000000000000000000 ) ) ;
#19478=CARTESIAN_POINT ( 'NONE',  ( -110.0000000000000142, 275.0000000000000000, 5.000000000000000888 ) ) ;
#19487=VERTEX_POINT ( 'NONE', #2548 ) ;
#19531=EDGE_LOOP ( 'NONE', ( #1161, #16500 ) ) ;
#19534=CARTESIAN_POINT ( 'NONE',  ( -189.9999999999988916, 285.0000000000000568, 12.50000000000027178 ) ) ;
#19559=FACE_OUTER_BOUND ( 'NONE', #16894, .T. ) ;
#19575=ORIENTED_EDGE ( 'NONE', *, *, #7007, .T. ) ;
#19661=CIRCLE ( 'NONE', #1036, 7.500000000000003553 ) ;
#19740=CIRCLE ( 'NONE', #13527, 99.99999999999997158 ) ;
#19747=DIRECTION ( 'NONE',  ( 0.000000000000000000, 0.000000000000000000, -1.000000000000000000 ) ) ;
#19759=SHAPE_REPRESENTATION_RELATIONSHIP ( 'NONE' , 'NONE' ,  #16185, #8694 ) ;
#19908=EDGE_LOOP ( 'NONE', ( #8020, #883, #11161, #638 ) ) ;
#19968=DIRECTION ( 'NONE',  ( 0.000000000000000000, 1.000000000000000000, 0.000000000000000000 ) ) ;
#20004=CARTESIAN_POINT ( 'NONE',  ( -29.99999999999887379, 275.0000000000000000, 4.999999999999158007 ) ) ;
#20024=DIRECTION ( 'NONE',  ( -0.000000000000000000, -1.000000000000000000, -0.000000000000000000 ) ) ;
#20034=DIRECTION ( 'NONE',  ( 0.000000000000000000, 1.000000000000000000, 0.000000000000000000 ) ) ;
#20121=DIRECTION ( 'NONE',  ( 0.000000000000000000, 0.000000000000000000, 1.000000000000000000 ) ) ;
#20156=DIRECTION ( 'NONE',  ( -0.000000000000000000, -1.000000000000000000, -0.000000000000000000 ) ) ;
#20192=AXIS2_PLACEMENT_3D ( 'NONE', #18571, #2618, #9044 ) ;
#20211=DIRECTION ( 'NONE',  ( 0.000000000000000000, 1.000000000000000000, 0.000000000000000000 ) ) ;
#20217=VECTOR ( 'NONE', #7221, 1000.000000000000000 ) ;
ENDSEC;
END-ISO-10303-21;
